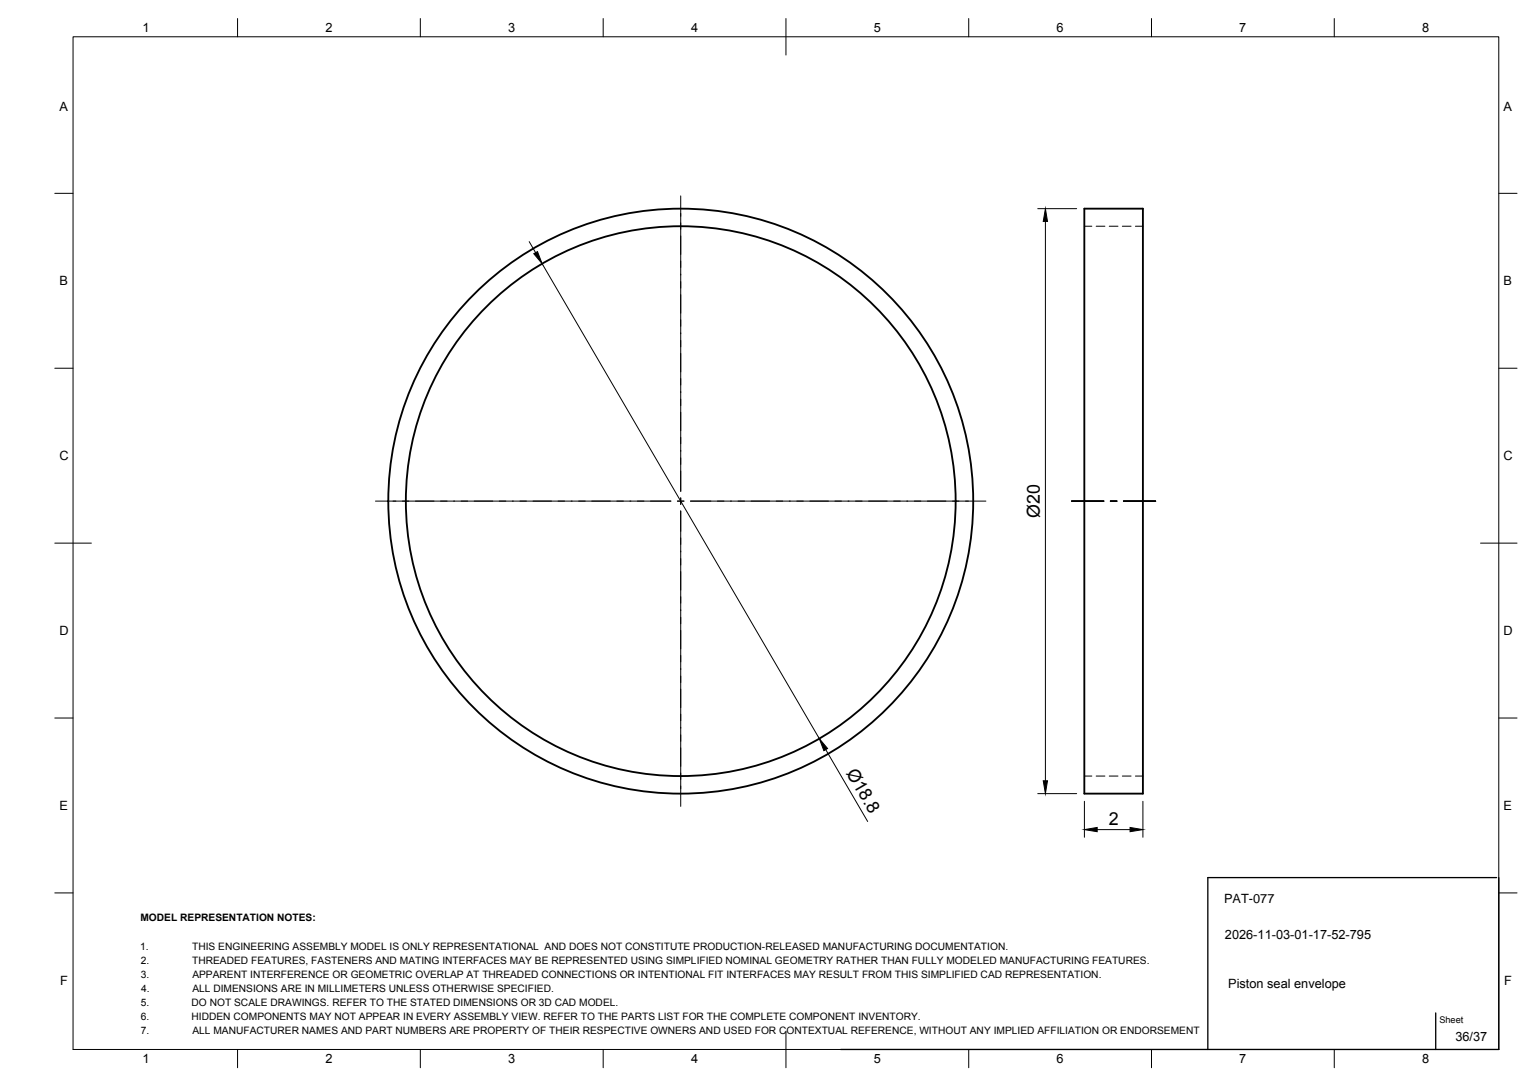
ISO-10303-21;
HEADER;
/* Generated by software containing ST-Developer
 * from STEP Tools, Inc. (www.steptools.com) 
 */

FILE_DESCRIPTION(
/* description */ ('Pallet stop with pneumatic fitting'),
/* implementation_level */ '2;1');

FILE_NAME(
/* name */ 'Piston seal envelope.step',
/* time_stamp */ '2026-10-27T10:51:41-07:00',
/* author */ (''),
/* organization */ (''),
/* preprocessor_version */ 'ST-DEVELOPER v20.2',
/* originating_system */ 'Autodesk Translation Framework v15.17.0.0',
/* authorisation */ '');

FILE_SCHEMA (('AUTOMOTIVE_DESIGN { 1 0 10303 214 3 1 1 }'));
ENDSEC;

DATA;
#10=MECHANICAL_DESIGN_GEOMETRIC_PRESENTATION_REPRESENTATION('',(#385),#10265);
#321=SHAPE_REPRESENTATION_RELATIONSHIP('SRR','None',#10437,#353);
#353=ADVANCED_BREP_SHAPE_REPRESENTATION('',(#416),#10261);
#385=STYLED_ITEM('',(#10662),#416);
#416=MANIFOLD_SOLID_BREP('Body1',#5074);
#541=FACE_BOUND('',#1453,.T.);
#542=FACE_BOUND('',#1455,.T.);
#712=PLANE('',#5982);
#713=PLANE('',#5983);
#1014=FACE_OUTER_BOUND('',#1450,.T.);
#1015=FACE_OUTER_BOUND('',#1451,.T.);
#1016=FACE_OUTER_BOUND('',#1452,.T.);
#1017=FACE_OUTER_BOUND('',#1454,.T.);
#1450=EDGE_LOOP('',(#4490,#4491,#4492,#4493));
#1451=EDGE_LOOP('',(#4494,#4495,#4496,#4497));
#1452=EDGE_LOOP('',(#4498));
#1453=EDGE_LOOP('',(#4499));
#1454=EDGE_LOOP('',(#4500));
#1455=EDGE_LOOP('',(#4501));
#1777=LINE('',#9991,#2112);
#1778=LINE('',#9997,#2113);
#2112=VECTOR('',#7468,0.94);
#2113=VECTOR('',#7475,1.);
#2389=CIRCLE('',#5977,0.94);
#2390=CIRCLE('',#5978,0.94);
#2391=CIRCLE('',#5980,1.);
#2392=CIRCLE('',#5981,1.);
#2762=VERTEX_POINT('',#9988);
#2763=VERTEX_POINT('',#9990);
#2764=VERTEX_POINT('',#9994);
#2765=VERTEX_POINT('',#9996);
#3344=EDGE_CURVE('',#2762,#2762,#2389,.T.);
#3345=EDGE_CURVE('',#2762,#2763,#1777,.T.);
#3346=EDGE_CURVE('',#2763,#2763,#2390,.T.);
#3347=EDGE_CURVE('',#2764,#2764,#2391,.T.);
#3348=EDGE_CURVE('',#2764,#2765,#1778,.T.);
#3349=EDGE_CURVE('',#2765,#2765,#2392,.T.);
#4490=ORIENTED_EDGE('',*,*,#3344,.F.);
#4491=ORIENTED_EDGE('',*,*,#3345,.T.);
#4492=ORIENTED_EDGE('',*,*,#3346,.T.);
#4493=ORIENTED_EDGE('',*,*,#3345,.F.);
#4494=ORIENTED_EDGE('',*,*,#3347,.F.);
#4495=ORIENTED_EDGE('',*,*,#3348,.T.);
#4496=ORIENTED_EDGE('',*,*,#3349,.T.);
#4497=ORIENTED_EDGE('',*,*,#3348,.F.);
#4498=ORIENTED_EDGE('',*,*,#3347,.T.);
#4499=ORIENTED_EDGE('',*,*,#3344,.T.);
#4500=ORIENTED_EDGE('',*,*,#3349,.F.);
#4501=ORIENTED_EDGE('',*,*,#3346,.F.);
#4725=CYLINDRICAL_SURFACE('',#5976,0.94);
#4726=CYLINDRICAL_SURFACE('',#5979,1.);
#5009=ADVANCED_FACE('',(#1014),#4725,.F.);
#5010=ADVANCED_FACE('',(#1015),#4726,.T.);
#5011=ADVANCED_FACE('',(#1016,#541),#712,.T.);
#5012=ADVANCED_FACE('',(#1017,#542),#713,.F.);
#5074=CLOSED_SHELL('',(#5009,#5010,#5011,#5012));
#5975=AXIS2_PLACEMENT_3D('',#9986,#7462,#7463);
#5976=AXIS2_PLACEMENT_3D('',#9987,#7464,#7465);
#5977=AXIS2_PLACEMENT_3D('',#9989,#7466,#7467);
#5978=AXIS2_PLACEMENT_3D('',#9992,#7469,#7470);
#5979=AXIS2_PLACEMENT_3D('',#9993,#7471,#7472);
#5980=AXIS2_PLACEMENT_3D('',#9995,#7473,#7474);
#5981=AXIS2_PLACEMENT_3D('',#9998,#7476,#7477);
#5982=AXIS2_PLACEMENT_3D('',#9999,#7478,#7479);
#5983=AXIS2_PLACEMENT_3D('',#10000,#7480,#7481);
#7462=DIRECTION('axis',(0.,0.,1.));
#7463=DIRECTION('refdir',(1.,0.,0.));
#7464=DIRECTION('center_axis',(0.,0.,1.));
#7465=DIRECTION('ref_axis',(1.,0.,0.));
#7466=DIRECTION('center_axis',(0.,0.,-1.));
#7467=DIRECTION('ref_axis',(1.,0.,0.));
#7468=DIRECTION('',(0.,0.,-1.));
#7469=DIRECTION('center_axis',(0.,0.,-1.));
#7470=DIRECTION('ref_axis',(1.,0.,0.));
#7471=DIRECTION('center_axis',(0.,0.,1.));
#7472=DIRECTION('ref_axis',(1.,0.,0.));
#7473=DIRECTION('center_axis',(0.,0.,1.));
#7474=DIRECTION('ref_axis',(1.,0.,0.));
#7475=DIRECTION('',(0.,0.,-1.));
#7476=DIRECTION('center_axis',(0.,0.,1.));
#7477=DIRECTION('ref_axis',(1.,0.,0.));
#7478=DIRECTION('center_axis',(0.,0.,1.));
#7479=DIRECTION('ref_axis',(1.,0.,0.));
#7480=DIRECTION('center_axis',(0.,0.,1.));
#7481=DIRECTION('ref_axis',(1.,0.,0.));
#9986=CARTESIAN_POINT('',(0.,0.,0.));
#9987=CARTESIAN_POINT('Origin',(4.,4.,7.3));
#9988=CARTESIAN_POINT('',(3.06,4.,7.5));
#9989=CARTESIAN_POINT('Origin',(4.,4.,7.5));
#9990=CARTESIAN_POINT('',(3.06,4.,7.3));
#9991=CARTESIAN_POINT('',(3.06,4.,7.3));
#9992=CARTESIAN_POINT('Origin',(4.,4.,7.3));
#9993=CARTESIAN_POINT('Origin',(4.,4.,7.3));
#9994=CARTESIAN_POINT('',(3.,4.,7.5));
#9995=CARTESIAN_POINT('Origin',(4.,4.,7.5));
#9996=CARTESIAN_POINT('',(3.,4.,7.3));
#9997=CARTESIAN_POINT('',(3.,4.,7.3));
#9998=CARTESIAN_POINT('Origin',(4.,4.,7.3));
#9999=CARTESIAN_POINT('Origin',(4.,4.,7.5));
#10000=CARTESIAN_POINT('Origin',(4.,4.,7.3));
#10223=UNCERTAINTY_MEASURE_WITH_UNIT(LENGTH_MEASURE(0.001),#10266,
'DISTANCE_ACCURACY_VALUE',
'Maximum model space distance between geometric entities at asserted c
onnectivities');
#10227=UNCERTAINTY_MEASURE_WITH_UNIT(LENGTH_MEASURE(0.001),#10266,
'DISTANCE_ACCURACY_VALUE',
'Maximum model space distance between geometric entities at asserted c
onnectivities');
#10261=(
GEOMETRIC_REPRESENTATION_CONTEXT(3)
GLOBAL_UNCERTAINTY_ASSIGNED_CONTEXT((#10223))
GLOBAL_UNIT_ASSIGNED_CONTEXT((#10266,#10268,#10269))
REPRESENTATION_CONTEXT('','3D')
);
#10265=(
GEOMETRIC_REPRESENTATION_CONTEXT(3)
GLOBAL_UNCERTAINTY_ASSIGNED_CONTEXT((#10227))
GLOBAL_UNIT_ASSIGNED_CONTEXT((#10266,#10268,#10269))
REPRESENTATION_CONTEXT('','3D')
);
#10266=(
LENGTH_UNIT()
NAMED_UNIT(*)
SI_UNIT(.CENTI.,.METRE.)
);
#10268=(
NAMED_UNIT(*)
PLANE_ANGLE_UNIT()
SI_UNIT($,.RADIAN.)
);
#10269=(
NAMED_UNIT(*)
SI_UNIT($,.STERADIAN.)
SOLID_ANGLE_UNIT()
);
#10303=SHAPE_DEFINITION_REPRESENTATION(#10344,#10437);
#10344=PRODUCT_DEFINITION_SHAPE('',$,#10475);
#10437=SHAPE_REPRESENTATION('',(#5975),#10261);
#10441=PRODUCT_DEFINITION_CONTEXT('part definition',#10554,'design');
#10475=PRODUCT_DEFINITION('Piston seal envelope','Piston seal envelope',
#10512,#10441);
#10512=PRODUCT_DEFINITION_FORMATION('',$,#10589);
#10554=APPLICATION_CONTEXT(
'Core Data for Automotive Mechanical Design Process');
#10555=PRODUCT_CONTEXT('part definition',#10554,'mechanical');
#10589=PRODUCT('Piston seal envelope','Piston seal envelope',
'Piston seal envelope',(#10555));
#10656=COLOUR_RGB('Black',0.12,0.14,0.17);
#10657=FILL_AREA_STYLE_COLOUR('',#10656);
#10658=FILL_AREA_STYLE('',(#10657));
#10659=SURFACE_STYLE_FILL_AREA(#10658);
#10660=SURFACE_SIDE_STYLE('',(#10659));
#10661=SURFACE_STYLE_USAGE(.BOTH.,#10660);
#10662=PRESENTATION_STYLE_ASSIGNMENT((#10661));
ENDSEC;
END-ISO-10303-21;
